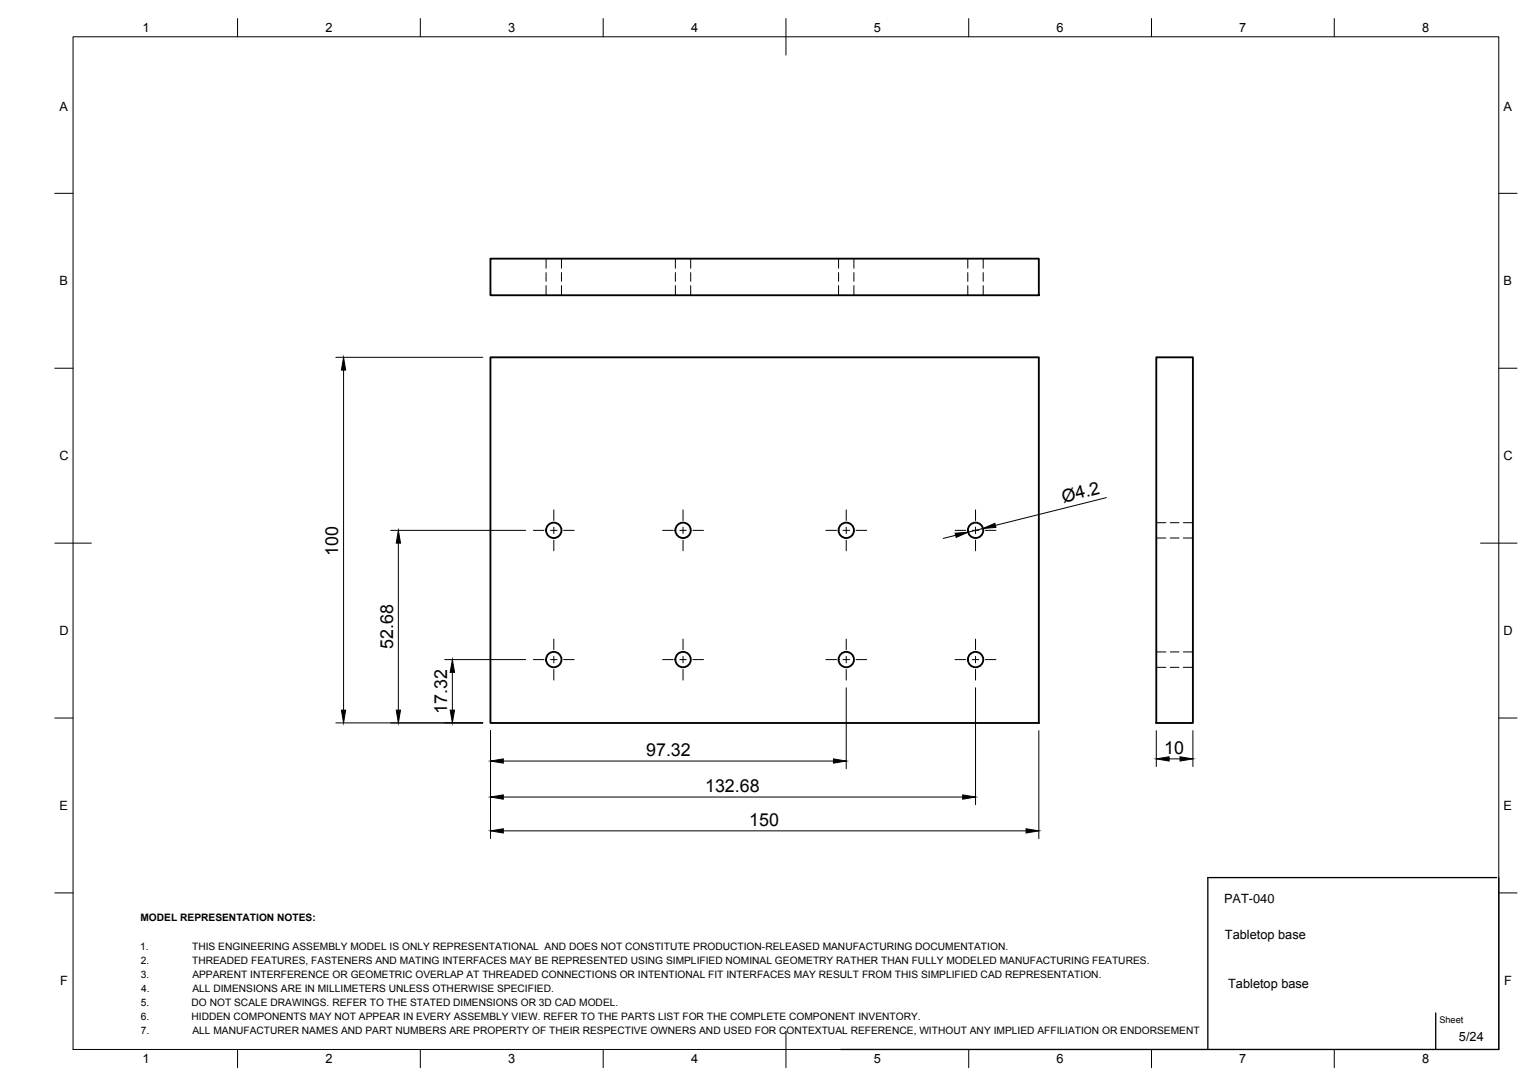
ISO-10303-21;
HEADER;
/* Generated by software containing ST-Developer
 * from STEP Tools, Inc. (www.steptools.com) 
 */

FILE_DESCRIPTION(
/* description */ ('Four-bar tabletop demonstrator'),
/* implementation_level */ '2;1');

FILE_NAME(
/* name */ 'Tabletop base.step',
/* time_stamp */ '2026-10-29T17:05:23-07:00',
/* author */ (''),
/* organization */ (''),
/* preprocessor_version */ 'ST-DEVELOPER v20.2',
/* originating_system */ 'Autodesk Translation Framework v15.17.0.0',
/* authorisation */ '');

FILE_SCHEMA (('AUTOMOTIVE_DESIGN { 1 0 10303 214 3 1 1 }'));
ENDSEC;

DATA;
#10=MECHANICAL_DESIGN_GEOMETRIC_PRESENTATION_REPRESENTATION('',(#337),#6705);
#307=SHAPE_REPRESENTATION_RELATIONSHIP('SRR','None',#6813,#322);
#322=ADVANCED_BREP_SHAPE_REPRESENTATION('',(#360),#6686);
#337=STYLED_ITEM('',(#6968),#360);
#360=MANIFOLD_SOLID_BREP('Body1',#3381);
#381=FACE_BOUND('',#778,.T.);
#382=FACE_BOUND('',#779,.T.);
#383=FACE_BOUND('',#780,.T.);
#384=FACE_BOUND('',#781,.T.);
#385=FACE_BOUND('',#782,.T.);
#386=FACE_BOUND('',#783,.T.);
#387=FACE_BOUND('',#784,.T.);
#388=FACE_BOUND('',#785,.T.);
#389=FACE_BOUND('',#787,.T.);
#390=FACE_BOUND('',#788,.T.);
#391=FACE_BOUND('',#789,.T.);
#392=FACE_BOUND('',#790,.T.);
#393=FACE_BOUND('',#791,.T.);
#394=FACE_BOUND('',#792,.T.);
#395=FACE_BOUND('',#793,.T.);
#396=FACE_BOUND('',#794,.T.);
#462=PLANE('',#3599);
#463=PLANE('',#3600);
#464=PLANE('',#3601);
#465=PLANE('',#3602);
#466=PLANE('',#3603);
#467=PLANE('',#3604);
#562=FACE_OUTER_BOUND('',#765,.T.);
#563=FACE_OUTER_BOUND('',#766,.T.);
#564=FACE_OUTER_BOUND('',#767,.T.);
#565=FACE_OUTER_BOUND('',#768,.T.);
#566=FACE_OUTER_BOUND('',#769,.T.);
#567=FACE_OUTER_BOUND('',#770,.T.);
#568=FACE_OUTER_BOUND('',#771,.T.);
#569=FACE_OUTER_BOUND('',#772,.T.);
#570=FACE_OUTER_BOUND('',#773,.T.);
#571=FACE_OUTER_BOUND('',#774,.T.);
#572=FACE_OUTER_BOUND('',#775,.T.);
#573=FACE_OUTER_BOUND('',#776,.T.);
#574=FACE_OUTER_BOUND('',#777,.T.);
#575=FACE_OUTER_BOUND('',#786,.T.);
#765=EDGE_LOOP('',(#2288,#2289,#2290,#2291));
#766=EDGE_LOOP('',(#2292,#2293,#2294,#2295));
#767=EDGE_LOOP('',(#2296,#2297,#2298,#2299));
#768=EDGE_LOOP('',(#2300,#2301,#2302,#2303));
#769=EDGE_LOOP('',(#2304,#2305,#2306,#2307));
#770=EDGE_LOOP('',(#2308,#2309,#2310,#2311));
#771=EDGE_LOOP('',(#2312,#2313,#2314,#2315));
#772=EDGE_LOOP('',(#2316,#2317,#2318,#2319));
#773=EDGE_LOOP('',(#2320,#2321,#2322,#2323));
#774=EDGE_LOOP('',(#2324,#2325,#2326,#2327));
#775=EDGE_LOOP('',(#2328,#2329,#2330,#2331));
#776=EDGE_LOOP('',(#2332,#2333,#2334,#2335));
#777=EDGE_LOOP('',(#2336,#2337,#2338,#2339));
#778=EDGE_LOOP('',(#2340));
#779=EDGE_LOOP('',(#2341));
#780=EDGE_LOOP('',(#2342));
#781=EDGE_LOOP('',(#2343));
#782=EDGE_LOOP('',(#2344));
#783=EDGE_LOOP('',(#2345));
#784=EDGE_LOOP('',(#2346));
#785=EDGE_LOOP('',(#2347));
#786=EDGE_LOOP('',(#2348,#2349,#2350,#2351));
#787=EDGE_LOOP('',(#2352));
#788=EDGE_LOOP('',(#2353));
#789=EDGE_LOOP('',(#2354));
#790=EDGE_LOOP('',(#2355));
#791=EDGE_LOOP('',(#2356));
#792=EDGE_LOOP('',(#2357));
#793=EDGE_LOOP('',(#2358));
#794=EDGE_LOOP('',(#2359));
#1049=LINE('',#5231,#1219);
#1050=LINE('',#5237,#1220);
#1051=LINE('',#5243,#1221);
#1052=LINE('',#5249,#1222);
#1053=LINE('',#5255,#1223);
#1054=LINE('',#5261,#1224);
#1055=LINE('',#5267,#1225);
#1056=LINE('',#5273,#1226);
#1057=LINE('',#5278,#1227);
#1058=LINE('',#5280,#1228);
#1059=LINE('',#5282,#1229);
#1060=LINE('',#5283,#1230);
#1061=LINE('',#5286,#1231);
#1062=LINE('',#5288,#1232);
#1063=LINE('',#5289,#1233);
#1064=LINE('',#5292,#1234);
#1065=LINE('',#5294,#1235);
#1066=LINE('',#5295,#1236);
#1067=LINE('',#5297,#1237);
#1068=LINE('',#5298,#1238);
#1219=VECTOR('',#4076,0.21);
#1220=VECTOR('',#4083,0.21);
#1221=VECTOR('',#4090,0.210000000000001);
#1222=VECTOR('',#4097,0.210000000000001);
#1223=VECTOR('',#4104,0.21);
#1224=VECTOR('',#4111,0.21);
#1225=VECTOR('',#4118,0.21);
#1226=VECTOR('',#4125,0.21);
#1227=VECTOR('',#4130,1.);
#1228=VECTOR('',#4131,1.);
#1229=VECTOR('',#4132,1.);
#1230=VECTOR('',#4133,1.);
#1231=VECTOR('',#4136,1.);
#1232=VECTOR('',#4137,1.);
#1233=VECTOR('',#4138,1.);
#1234=VECTOR('',#4141,1.);
#1235=VECTOR('',#4142,1.);
#1236=VECTOR('',#4143,1.);
#1237=VECTOR('',#4146,1.);
#1238=VECTOR('',#4147,1.);
#1389=CIRCLE('',#3576,0.21);
#1390=CIRCLE('',#3577,0.21);
#1391=CIRCLE('',#3579,0.21);
#1392=CIRCLE('',#3580,0.21);
#1393=CIRCLE('',#3582,0.210000000000001);
#1394=CIRCLE('',#3583,0.210000000000001);
#1395=CIRCLE('',#3585,0.210000000000001);
#1396=CIRCLE('',#3586,0.210000000000001);
#1397=CIRCLE('',#3588,0.21);
#1398=CIRCLE('',#3589,0.21);
#1399=CIRCLE('',#3591,0.21);
#1400=CIRCLE('',#3592,0.21);
#1401=CIRCLE('',#3594,0.21);
#1402=CIRCLE('',#3595,0.21);
#1403=CIRCLE('',#3597,0.21);
#1404=CIRCLE('',#3598,0.21);
#1600=VERTEX_POINT('',#5228);
#1601=VERTEX_POINT('',#5230);
#1602=VERTEX_POINT('',#5234);
#1603=VERTEX_POINT('',#5236);
#1604=VERTEX_POINT('',#5240);
#1605=VERTEX_POINT('',#5242);
#1606=VERTEX_POINT('',#5246);
#1607=VERTEX_POINT('',#5248);
#1608=VERTEX_POINT('',#5252);
#1609=VERTEX_POINT('',#5254);
#1610=VERTEX_POINT('',#5258);
#1611=VERTEX_POINT('',#5260);
#1612=VERTEX_POINT('',#5264);
#1613=VERTEX_POINT('',#5266);
#1614=VERTEX_POINT('',#5270);
#1615=VERTEX_POINT('',#5272);
#1616=VERTEX_POINT('',#5276);
#1617=VERTEX_POINT('',#5277);
#1618=VERTEX_POINT('',#5279);
#1619=VERTEX_POINT('',#5281);
#1620=VERTEX_POINT('',#5285);
#1621=VERTEX_POINT('',#5287);
#1622=VERTEX_POINT('',#5291);
#1623=VERTEX_POINT('',#5293);
#1880=EDGE_CURVE('',#1600,#1600,#1389,.T.);
#1881=EDGE_CURVE('',#1600,#1601,#1049,.T.);
#1882=EDGE_CURVE('',#1601,#1601,#1390,.T.);
#1883=EDGE_CURVE('',#1602,#1602,#1391,.T.);
#1884=EDGE_CURVE('',#1602,#1603,#1050,.T.);
#1885=EDGE_CURVE('',#1603,#1603,#1392,.T.);
#1886=EDGE_CURVE('',#1604,#1604,#1393,.T.);
#1887=EDGE_CURVE('',#1604,#1605,#1051,.T.);
#1888=EDGE_CURVE('',#1605,#1605,#1394,.T.);
#1889=EDGE_CURVE('',#1606,#1606,#1395,.T.);
#1890=EDGE_CURVE('',#1606,#1607,#1052,.T.);
#1891=EDGE_CURVE('',#1607,#1607,#1396,.T.);
#1892=EDGE_CURVE('',#1608,#1608,#1397,.T.);
#1893=EDGE_CURVE('',#1608,#1609,#1053,.T.);
#1894=EDGE_CURVE('',#1609,#1609,#1398,.T.);
#1895=EDGE_CURVE('',#1610,#1610,#1399,.T.);
#1896=EDGE_CURVE('',#1610,#1611,#1054,.T.);
#1897=EDGE_CURVE('',#1611,#1611,#1400,.T.);
#1898=EDGE_CURVE('',#1612,#1612,#1401,.T.);
#1899=EDGE_CURVE('',#1612,#1613,#1055,.T.);
#1900=EDGE_CURVE('',#1613,#1613,#1402,.T.);
#1901=EDGE_CURVE('',#1614,#1614,#1403,.T.);
#1902=EDGE_CURVE('',#1614,#1615,#1056,.T.);
#1903=EDGE_CURVE('',#1615,#1615,#1404,.T.);
#1904=EDGE_CURVE('',#1616,#1617,#1057,.T.);
#1905=EDGE_CURVE('',#1617,#1618,#1058,.T.);
#1906=EDGE_CURVE('',#1619,#1618,#1059,.T.);
#1907=EDGE_CURVE('',#1616,#1619,#1060,.T.);
#1908=EDGE_CURVE('',#1620,#1616,#1061,.T.);
#1909=EDGE_CURVE('',#1621,#1619,#1062,.T.);
#1910=EDGE_CURVE('',#1620,#1621,#1063,.T.);
#1911=EDGE_CURVE('',#1622,#1620,#1064,.T.);
#1912=EDGE_CURVE('',#1623,#1621,#1065,.T.);
#1913=EDGE_CURVE('',#1622,#1623,#1066,.T.);
#1914=EDGE_CURVE('',#1617,#1622,#1067,.T.);
#1915=EDGE_CURVE('',#1618,#1623,#1068,.T.);
#2288=ORIENTED_EDGE('',*,*,#1880,.F.);
#2289=ORIENTED_EDGE('',*,*,#1881,.T.);
#2290=ORIENTED_EDGE('',*,*,#1882,.F.);
#2291=ORIENTED_EDGE('',*,*,#1881,.F.);
#2292=ORIENTED_EDGE('',*,*,#1883,.F.);
#2293=ORIENTED_EDGE('',*,*,#1884,.T.);
#2294=ORIENTED_EDGE('',*,*,#1885,.F.);
#2295=ORIENTED_EDGE('',*,*,#1884,.F.);
#2296=ORIENTED_EDGE('',*,*,#1886,.F.);
#2297=ORIENTED_EDGE('',*,*,#1887,.T.);
#2298=ORIENTED_EDGE('',*,*,#1888,.F.);
#2299=ORIENTED_EDGE('',*,*,#1887,.F.);
#2300=ORIENTED_EDGE('',*,*,#1889,.F.);
#2301=ORIENTED_EDGE('',*,*,#1890,.T.);
#2302=ORIENTED_EDGE('',*,*,#1891,.F.);
#2303=ORIENTED_EDGE('',*,*,#1890,.F.);
#2304=ORIENTED_EDGE('',*,*,#1892,.F.);
#2305=ORIENTED_EDGE('',*,*,#1893,.T.);
#2306=ORIENTED_EDGE('',*,*,#1894,.F.);
#2307=ORIENTED_EDGE('',*,*,#1893,.F.);
#2308=ORIENTED_EDGE('',*,*,#1895,.F.);
#2309=ORIENTED_EDGE('',*,*,#1896,.T.);
#2310=ORIENTED_EDGE('',*,*,#1897,.F.);
#2311=ORIENTED_EDGE('',*,*,#1896,.F.);
#2312=ORIENTED_EDGE('',*,*,#1898,.F.);
#2313=ORIENTED_EDGE('',*,*,#1899,.T.);
#2314=ORIENTED_EDGE('',*,*,#1900,.F.);
#2315=ORIENTED_EDGE('',*,*,#1899,.F.);
#2316=ORIENTED_EDGE('',*,*,#1901,.F.);
#2317=ORIENTED_EDGE('',*,*,#1902,.T.);
#2318=ORIENTED_EDGE('',*,*,#1903,.F.);
#2319=ORIENTED_EDGE('',*,*,#1902,.F.);
#2320=ORIENTED_EDGE('',*,*,#1904,.T.);
#2321=ORIENTED_EDGE('',*,*,#1905,.T.);
#2322=ORIENTED_EDGE('',*,*,#1906,.F.);
#2323=ORIENTED_EDGE('',*,*,#1907,.F.);
#2324=ORIENTED_EDGE('',*,*,#1908,.T.);
#2325=ORIENTED_EDGE('',*,*,#1907,.T.);
#2326=ORIENTED_EDGE('',*,*,#1909,.F.);
#2327=ORIENTED_EDGE('',*,*,#1910,.F.);
#2328=ORIENTED_EDGE('',*,*,#1911,.T.);
#2329=ORIENTED_EDGE('',*,*,#1910,.T.);
#2330=ORIENTED_EDGE('',*,*,#1912,.F.);
#2331=ORIENTED_EDGE('',*,*,#1913,.F.);
#2332=ORIENTED_EDGE('',*,*,#1914,.T.);
#2333=ORIENTED_EDGE('',*,*,#1913,.T.);
#2334=ORIENTED_EDGE('',*,*,#1915,.F.);
#2335=ORIENTED_EDGE('',*,*,#1905,.F.);
#2336=ORIENTED_EDGE('',*,*,#1915,.T.);
#2337=ORIENTED_EDGE('',*,*,#1912,.T.);
#2338=ORIENTED_EDGE('',*,*,#1909,.T.);
#2339=ORIENTED_EDGE('',*,*,#1906,.T.);
#2340=ORIENTED_EDGE('',*,*,#1903,.T.);
#2341=ORIENTED_EDGE('',*,*,#1900,.T.);
#2342=ORIENTED_EDGE('',*,*,#1897,.T.);
#2343=ORIENTED_EDGE('',*,*,#1894,.T.);
#2344=ORIENTED_EDGE('',*,*,#1891,.T.);
#2345=ORIENTED_EDGE('',*,*,#1888,.T.);
#2346=ORIENTED_EDGE('',*,*,#1885,.T.);
#2347=ORIENTED_EDGE('',*,*,#1882,.T.);
#2348=ORIENTED_EDGE('',*,*,#1914,.F.);
#2349=ORIENTED_EDGE('',*,*,#1904,.F.);
#2350=ORIENTED_EDGE('',*,*,#1908,.F.);
#2351=ORIENTED_EDGE('',*,*,#1911,.F.);
#2352=ORIENTED_EDGE('',*,*,#1901,.T.);
#2353=ORIENTED_EDGE('',*,*,#1898,.T.);
#2354=ORIENTED_EDGE('',*,*,#1895,.T.);
#2355=ORIENTED_EDGE('',*,*,#1892,.T.);
#2356=ORIENTED_EDGE('',*,*,#1889,.T.);
#2357=ORIENTED_EDGE('',*,*,#1886,.T.);
#2358=ORIENTED_EDGE('',*,*,#1883,.T.);
#2359=ORIENTED_EDGE('',*,*,#1880,.T.);
#3104=CYLINDRICAL_SURFACE('',#3575,0.21);
#3105=CYLINDRICAL_SURFACE('',#3578,0.21);
#3106=CYLINDRICAL_SURFACE('',#3581,0.210000000000001);
#3107=CYLINDRICAL_SURFACE('',#3584,0.210000000000001);
#3108=CYLINDRICAL_SURFACE('',#3587,0.21);
#3109=CYLINDRICAL_SURFACE('',#3590,0.21);
#3110=CYLINDRICAL_SURFACE('',#3593,0.21);
#3111=CYLINDRICAL_SURFACE('',#3596,0.21);
#3178=ADVANCED_FACE('',(#562),#3104,.F.);
#3179=ADVANCED_FACE('',(#563),#3105,.F.);
#3180=ADVANCED_FACE('',(#564),#3106,.F.);
#3181=ADVANCED_FACE('',(#565),#3107,.F.);
#3182=ADVANCED_FACE('',(#566),#3108,.F.);
#3183=ADVANCED_FACE('',(#567),#3109,.F.);
#3184=ADVANCED_FACE('',(#568),#3110,.F.);
#3185=ADVANCED_FACE('',(#569),#3111,.F.);
#3186=ADVANCED_FACE('',(#570),#462,.T.);
#3187=ADVANCED_FACE('',(#571),#463,.T.);
#3188=ADVANCED_FACE('',(#572),#464,.T.);
#3189=ADVANCED_FACE('',(#573),#465,.T.);
#3190=ADVANCED_FACE('',(#574,#381,#382,#383,#384,#385,#386,#387,#388),#466,
 .T.);
#3191=ADVANCED_FACE('',(#575,#389,#390,#391,#392,#393,#394,#395,#396),#467,
 .F.);
#3381=CLOSED_SHELL('',(#3178,#3179,#3180,#3181,#3182,#3183,#3184,#3185,
#3186,#3187,#3188,#3189,#3190,#3191));
#3574=AXIS2_PLACEMENT_3D('',#5226,#4070,#4071);
#3575=AXIS2_PLACEMENT_3D('',#5227,#4072,#4073);
#3576=AXIS2_PLACEMENT_3D('',#5229,#4074,#4075);
#3577=AXIS2_PLACEMENT_3D('',#5232,#4077,#4078);
#3578=AXIS2_PLACEMENT_3D('',#5233,#4079,#4080);
#3579=AXIS2_PLACEMENT_3D('',#5235,#4081,#4082);
#3580=AXIS2_PLACEMENT_3D('',#5238,#4084,#4085);
#3581=AXIS2_PLACEMENT_3D('',#5239,#4086,#4087);
#3582=AXIS2_PLACEMENT_3D('',#5241,#4088,#4089);
#3583=AXIS2_PLACEMENT_3D('',#5244,#4091,#4092);
#3584=AXIS2_PLACEMENT_3D('',#5245,#4093,#4094);
#3585=AXIS2_PLACEMENT_3D('',#5247,#4095,#4096);
#3586=AXIS2_PLACEMENT_3D('',#5250,#4098,#4099);
#3587=AXIS2_PLACEMENT_3D('',#5251,#4100,#4101);
#3588=AXIS2_PLACEMENT_3D('',#5253,#4102,#4103);
#3589=AXIS2_PLACEMENT_3D('',#5256,#4105,#4106);
#3590=AXIS2_PLACEMENT_3D('',#5257,#4107,#4108);
#3591=AXIS2_PLACEMENT_3D('',#5259,#4109,#4110);
#3592=AXIS2_PLACEMENT_3D('',#5262,#4112,#4113);
#3593=AXIS2_PLACEMENT_3D('',#5263,#4114,#4115);
#3594=AXIS2_PLACEMENT_3D('',#5265,#4116,#4117);
#3595=AXIS2_PLACEMENT_3D('',#5268,#4119,#4120);
#3596=AXIS2_PLACEMENT_3D('',#5269,#4121,#4122);
#3597=AXIS2_PLACEMENT_3D('',#5271,#4123,#4124);
#3598=AXIS2_PLACEMENT_3D('',#5274,#4126,#4127);
#3599=AXIS2_PLACEMENT_3D('',#5275,#4128,#4129);
#3600=AXIS2_PLACEMENT_3D('',#5284,#4134,#4135);
#3601=AXIS2_PLACEMENT_3D('',#5290,#4139,#4140);
#3602=AXIS2_PLACEMENT_3D('',#5296,#4144,#4145);
#3603=AXIS2_PLACEMENT_3D('',#5299,#4148,#4149);
#3604=AXIS2_PLACEMENT_3D('',#5300,#4150,#4151);
#4070=DIRECTION('axis',(0.,0.,1.));
#4071=DIRECTION('refdir',(1.,0.,0.));
#4072=DIRECTION('center_axis',(0.,0.,1.));
#4073=DIRECTION('ref_axis',(1.,0.,0.));
#4074=DIRECTION('center_axis',(0.,0.,1.));
#4075=DIRECTION('ref_axis',(1.,0.,0.));
#4076=DIRECTION('',(0.,0.,1.));
#4077=DIRECTION('center_axis',(0.,0.,-1.));
#4078=DIRECTION('ref_axis',(1.,0.,0.));
#4079=DIRECTION('center_axis',(0.,0.,1.));
#4080=DIRECTION('ref_axis',(1.,0.,0.));
#4081=DIRECTION('center_axis',(0.,0.,1.));
#4082=DIRECTION('ref_axis',(1.,0.,0.));
#4083=DIRECTION('',(0.,0.,1.));
#4084=DIRECTION('center_axis',(0.,0.,-1.));
#4085=DIRECTION('ref_axis',(1.,0.,0.));
#4086=DIRECTION('center_axis',(0.,0.,1.));
#4087=DIRECTION('ref_axis',(1.,0.,0.));
#4088=DIRECTION('center_axis',(0.,0.,1.));
#4089=DIRECTION('ref_axis',(1.,0.,0.));
#4090=DIRECTION('',(0.,0.,1.));
#4091=DIRECTION('center_axis',(0.,0.,-1.));
#4092=DIRECTION('ref_axis',(1.,0.,0.));
#4093=DIRECTION('center_axis',(0.,0.,1.));
#4094=DIRECTION('ref_axis',(1.,0.,0.));
#4095=DIRECTION('center_axis',(0.,0.,1.));
#4096=DIRECTION('ref_axis',(1.,0.,0.));
#4097=DIRECTION('',(0.,0.,1.));
#4098=DIRECTION('center_axis',(0.,0.,-1.));
#4099=DIRECTION('ref_axis',(1.,0.,0.));
#4100=DIRECTION('center_axis',(0.,0.,1.));
#4101=DIRECTION('ref_axis',(1.,0.,0.));
#4102=DIRECTION('center_axis',(0.,0.,1.));
#4103=DIRECTION('ref_axis',(1.,0.,0.));
#4104=DIRECTION('',(0.,0.,1.));
#4105=DIRECTION('center_axis',(0.,0.,-1.));
#4106=DIRECTION('ref_axis',(1.,0.,0.));
#4107=DIRECTION('center_axis',(0.,0.,1.));
#4108=DIRECTION('ref_axis',(1.,0.,0.));
#4109=DIRECTION('center_axis',(0.,0.,1.));
#4110=DIRECTION('ref_axis',(1.,0.,0.));
#4111=DIRECTION('',(0.,0.,1.));
#4112=DIRECTION('center_axis',(0.,0.,-1.));
#4113=DIRECTION('ref_axis',(1.,0.,0.));
#4114=DIRECTION('center_axis',(0.,0.,1.));
#4115=DIRECTION('ref_axis',(1.,0.,0.));
#4116=DIRECTION('center_axis',(0.,0.,1.));
#4117=DIRECTION('ref_axis',(1.,0.,0.));
#4118=DIRECTION('',(0.,0.,1.));
#4119=DIRECTION('center_axis',(0.,0.,-1.));
#4120=DIRECTION('ref_axis',(1.,0.,0.));
#4121=DIRECTION('center_axis',(0.,0.,1.));
#4122=DIRECTION('ref_axis',(1.,0.,0.));
#4123=DIRECTION('center_axis',(0.,0.,1.));
#4124=DIRECTION('ref_axis',(1.,0.,0.));
#4125=DIRECTION('',(0.,0.,1.));
#4126=DIRECTION('center_axis',(0.,0.,-1.));
#4127=DIRECTION('ref_axis',(1.,0.,0.));
#4128=DIRECTION('center_axis',(0.,1.,0.));
#4129=DIRECTION('ref_axis',(-1.,0.,0.));
#4130=DIRECTION('',(-1.,0.,0.));
#4131=DIRECTION('',(0.,0.,1.));
#4132=DIRECTION('',(-1.,0.,0.));
#4133=DIRECTION('',(0.,0.,1.));
#4134=DIRECTION('center_axis',(1.,0.,0.));
#4135=DIRECTION('ref_axis',(0.,1.,0.));
#4136=DIRECTION('',(0.,1.,0.));
#4137=DIRECTION('',(0.,1.,0.));
#4138=DIRECTION('',(0.,0.,1.));
#4139=DIRECTION('center_axis',(0.,-1.,0.));
#4140=DIRECTION('ref_axis',(1.,0.,0.));
#4141=DIRECTION('',(1.,0.,0.));
#4142=DIRECTION('',(1.,0.,0.));
#4143=DIRECTION('',(0.,0.,1.));
#4144=DIRECTION('center_axis',(-1.,0.,0.));
#4145=DIRECTION('ref_axis',(0.,-1.,0.));
#4146=DIRECTION('',(0.,-1.,0.));
#4147=DIRECTION('',(0.,-1.,0.));
#4148=DIRECTION('center_axis',(0.,0.,1.));
#4149=DIRECTION('ref_axis',(1.,0.,0.));
#4150=DIRECTION('center_axis',(0.,0.,1.));
#4151=DIRECTION('ref_axis',(1.,0.,0.));
#5226=CARTESIAN_POINT('',(0.,0.,0.));
#5227=CARTESIAN_POINT('Origin',(6.23223304703363,-1.76776695296637,-0.1));
#5228=CARTESIAN_POINT('',(6.02223304703363,-1.76776695296637,0.));
#5229=CARTESIAN_POINT('Origin',(6.23223304703363,-1.76776695296637,0.));
#5230=CARTESIAN_POINT('',(6.02223304703363,-1.76776695296637,1.));
#5231=CARTESIAN_POINT('',(6.02223304703363,-1.76776695296637,-0.1));
#5232=CARTESIAN_POINT('Origin',(6.23223304703363,-1.76776695296637,1.));
#5233=CARTESIAN_POINT('Origin',(6.23223304703363,1.76776695296637,-0.1));
#5234=CARTESIAN_POINT('',(6.02223304703363,1.76776695296637,0.));
#5235=CARTESIAN_POINT('Origin',(6.23223304703363,1.76776695296637,0.));
#5236=CARTESIAN_POINT('',(6.02223304703363,1.76776695296637,1.));
#5237=CARTESIAN_POINT('',(6.02223304703363,1.76776695296637,-0.1));
#5238=CARTESIAN_POINT('Origin',(6.23223304703363,1.76776695296637,1.));
#5239=CARTESIAN_POINT('Origin',(9.76776695296637,1.76776695296637,-0.1));
#5240=CARTESIAN_POINT('',(9.55776695296637,1.76776695296637,0.));
#5241=CARTESIAN_POINT('Origin',(9.76776695296637,1.76776695296637,0.));
#5242=CARTESIAN_POINT('',(9.55776695296637,1.76776695296637,1.));
#5243=CARTESIAN_POINT('',(9.55776695296637,1.76776695296637,-0.1));
#5244=CARTESIAN_POINT('Origin',(9.76776695296637,1.76776695296637,1.));
#5245=CARTESIAN_POINT('Origin',(9.76776695296637,-1.76776695296637,-0.1));
#5246=CARTESIAN_POINT('',(9.55776695296637,-1.76776695296637,0.));
#5247=CARTESIAN_POINT('Origin',(9.76776695296637,-1.76776695296637,0.));
#5248=CARTESIAN_POINT('',(9.55776695296637,-1.76776695296637,1.));
#5249=CARTESIAN_POINT('',(9.55776695296637,-1.76776695296637,-0.1));
#5250=CARTESIAN_POINT('Origin',(9.76776695296637,-1.76776695296637,1.));
#5251=CARTESIAN_POINT('Origin',(-1.76776695296637,-1.76776695296637,-0.1));
#5252=CARTESIAN_POINT('',(-1.97776695296637,-1.76776695296637,0.));
#5253=CARTESIAN_POINT('Origin',(-1.76776695296637,-1.76776695296637,0.));
#5254=CARTESIAN_POINT('',(-1.97776695296637,-1.76776695296637,1.));
#5255=CARTESIAN_POINT('',(-1.97776695296637,-1.76776695296637,-0.1));
#5256=CARTESIAN_POINT('Origin',(-1.76776695296637,-1.76776695296637,1.));
#5257=CARTESIAN_POINT('Origin',(-1.76776695296637,1.76776695296637,-0.1));
#5258=CARTESIAN_POINT('',(-1.97776695296637,1.76776695296637,0.));
#5259=CARTESIAN_POINT('Origin',(-1.76776695296637,1.76776695296637,0.));
#5260=CARTESIAN_POINT('',(-1.97776695296637,1.76776695296637,1.));
#5261=CARTESIAN_POINT('',(-1.97776695296637,1.76776695296637,-0.1));
#5262=CARTESIAN_POINT('Origin',(-1.76776695296637,1.76776695296637,1.));
#5263=CARTESIAN_POINT('Origin',(1.76776695296637,1.76776695296637,-0.1));
#5264=CARTESIAN_POINT('',(1.55776695296637,1.76776695296637,0.));
#5265=CARTESIAN_POINT('Origin',(1.76776695296637,1.76776695296637,0.));
#5266=CARTESIAN_POINT('',(1.55776695296637,1.76776695296637,1.));
#5267=CARTESIAN_POINT('',(1.55776695296637,1.76776695296637,-0.1));
#5268=CARTESIAN_POINT('Origin',(1.76776695296637,1.76776695296637,1.));
#5269=CARTESIAN_POINT('Origin',(1.76776695296637,-1.76776695296637,-0.1));
#5270=CARTESIAN_POINT('',(1.55776695296637,-1.76776695296637,0.));
#5271=CARTESIAN_POINT('Origin',(1.76776695296637,-1.76776695296637,0.));
#5272=CARTESIAN_POINT('',(1.55776695296637,-1.76776695296637,1.));
#5273=CARTESIAN_POINT('',(1.55776695296637,-1.76776695296637,-0.1));
#5274=CARTESIAN_POINT('Origin',(1.76776695296637,-1.76776695296637,1.));
#5275=CARTESIAN_POINT('Origin',(11.5,6.5,0.));
#5276=CARTESIAN_POINT('',(11.5,6.5,0.));
#5277=CARTESIAN_POINT('',(-3.5,6.5,0.));
#5278=CARTESIAN_POINT('',(11.5,6.5,0.));
#5279=CARTESIAN_POINT('',(-3.5,6.5,1.));
#5280=CARTESIAN_POINT('',(-3.5,6.5,0.));
#5281=CARTESIAN_POINT('',(11.5,6.5,1.));
#5282=CARTESIAN_POINT('',(11.5,6.5,1.));
#5283=CARTESIAN_POINT('',(11.5,6.5,0.));
#5284=CARTESIAN_POINT('Origin',(11.5,-3.5,0.));
#5285=CARTESIAN_POINT('',(11.5,-3.5,0.));
#5286=CARTESIAN_POINT('',(11.5,-3.5,0.));
#5287=CARTESIAN_POINT('',(11.5,-3.5,1.));
#5288=CARTESIAN_POINT('',(11.5,-3.5,1.));
#5289=CARTESIAN_POINT('',(11.5,-3.5,0.));
#5290=CARTESIAN_POINT('Origin',(-3.5,-3.5,0.));
#5291=CARTESIAN_POINT('',(-3.5,-3.5,0.));
#5292=CARTESIAN_POINT('',(-3.5,-3.5,0.));
#5293=CARTESIAN_POINT('',(-3.5,-3.5,1.));
#5294=CARTESIAN_POINT('',(-3.5,-3.5,1.));
#5295=CARTESIAN_POINT('',(-3.5,-3.5,0.));
#5296=CARTESIAN_POINT('Origin',(-3.5,6.5,0.));
#5297=CARTESIAN_POINT('',(-3.5,6.5,0.));
#5298=CARTESIAN_POINT('',(-3.5,6.5,1.));
#5299=CARTESIAN_POINT('Origin',(4.,1.5,1.));
#5300=CARTESIAN_POINT('Origin',(4.,1.5,0.));
#6664=UNCERTAINTY_MEASURE_WITH_UNIT(LENGTH_MEASURE(0.001),#6706,
'DISTANCE_ACCURACY_VALUE',
'Maximum model space distance between geometric entities at asserted c
onnectivities');
#6683=UNCERTAINTY_MEASURE_WITH_UNIT(LENGTH_MEASURE(0.001),#6706,
'DISTANCE_ACCURACY_VALUE',
'Maximum model space distance between geometric entities at asserted c
onnectivities');
#6686=(
GEOMETRIC_REPRESENTATION_CONTEXT(3)
GLOBAL_UNCERTAINTY_ASSIGNED_CONTEXT((#6664))
GLOBAL_UNIT_ASSIGNED_CONTEXT((#6706,#6708,#6709))
REPRESENTATION_CONTEXT('','3D')
);
#6705=(
GEOMETRIC_REPRESENTATION_CONTEXT(3)
GLOBAL_UNCERTAINTY_ASSIGNED_CONTEXT((#6683))
GLOBAL_UNIT_ASSIGNED_CONTEXT((#6706,#6708,#6709))
REPRESENTATION_CONTEXT('','3D')
);
#6706=(
LENGTH_UNIT()
NAMED_UNIT(*)
SI_UNIT(.CENTI.,.METRE.)
);
#6708=(
NAMED_UNIT(*)
PLANE_ANGLE_UNIT()
SI_UNIT($,.RADIAN.)
);
#6709=(
NAMED_UNIT(*)
SI_UNIT($,.STERADIAN.)
SOLID_ANGLE_UNIT()
);
#6712=SHAPE_DEFINITION_REPRESENTATION(#6733,#6813);
#6733=PRODUCT_DEFINITION_SHAPE('',$,#6835);
#6813=SHAPE_REPRESENTATION('',(#3574),#6686);
#6832=PRODUCT_DEFINITION_CONTEXT('part definition',#6897,'design');
#6835=PRODUCT_DEFINITION('Tabletop base','Tabletop base',#6856,#6832);
#6856=PRODUCT_DEFINITION_FORMATION('',$,#6901);
#6897=APPLICATION_CONTEXT(
'Core Data for Automotive Mechanical Design Process');
#6898=PRODUCT_CONTEXT('part definition',#6897,'mechanical');
#6901=PRODUCT('Tabletop base','Tabletop base','Tabletop base',(#6898));
#6962=COLOUR_RGB('Dark Blue',0.08,0.2,0.34);
#6963=FILL_AREA_STYLE_COLOUR('',#6962);
#6964=FILL_AREA_STYLE('',(#6963));
#6965=SURFACE_STYLE_FILL_AREA(#6964);
#6966=SURFACE_SIDE_STYLE('',(#6965));
#6967=SURFACE_STYLE_USAGE(.BOTH.,#6966);
#6968=PRESENTATION_STYLE_ASSIGNMENT((#6967));
ENDSEC;
END-ISO-10303-21;
